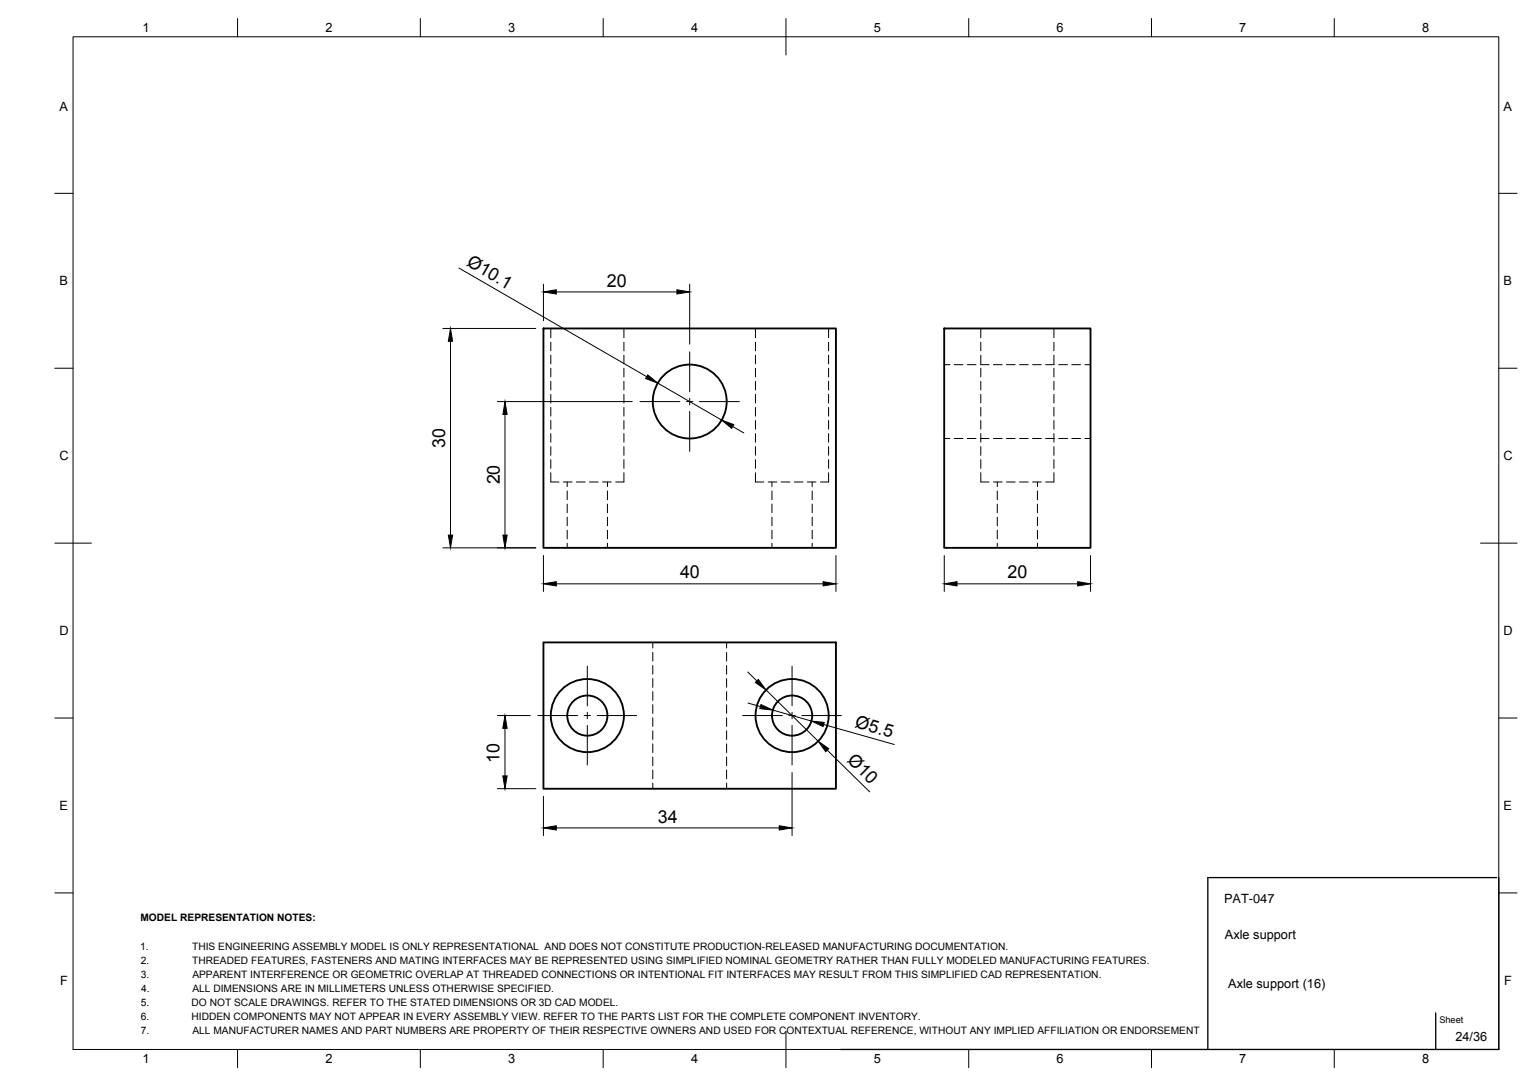
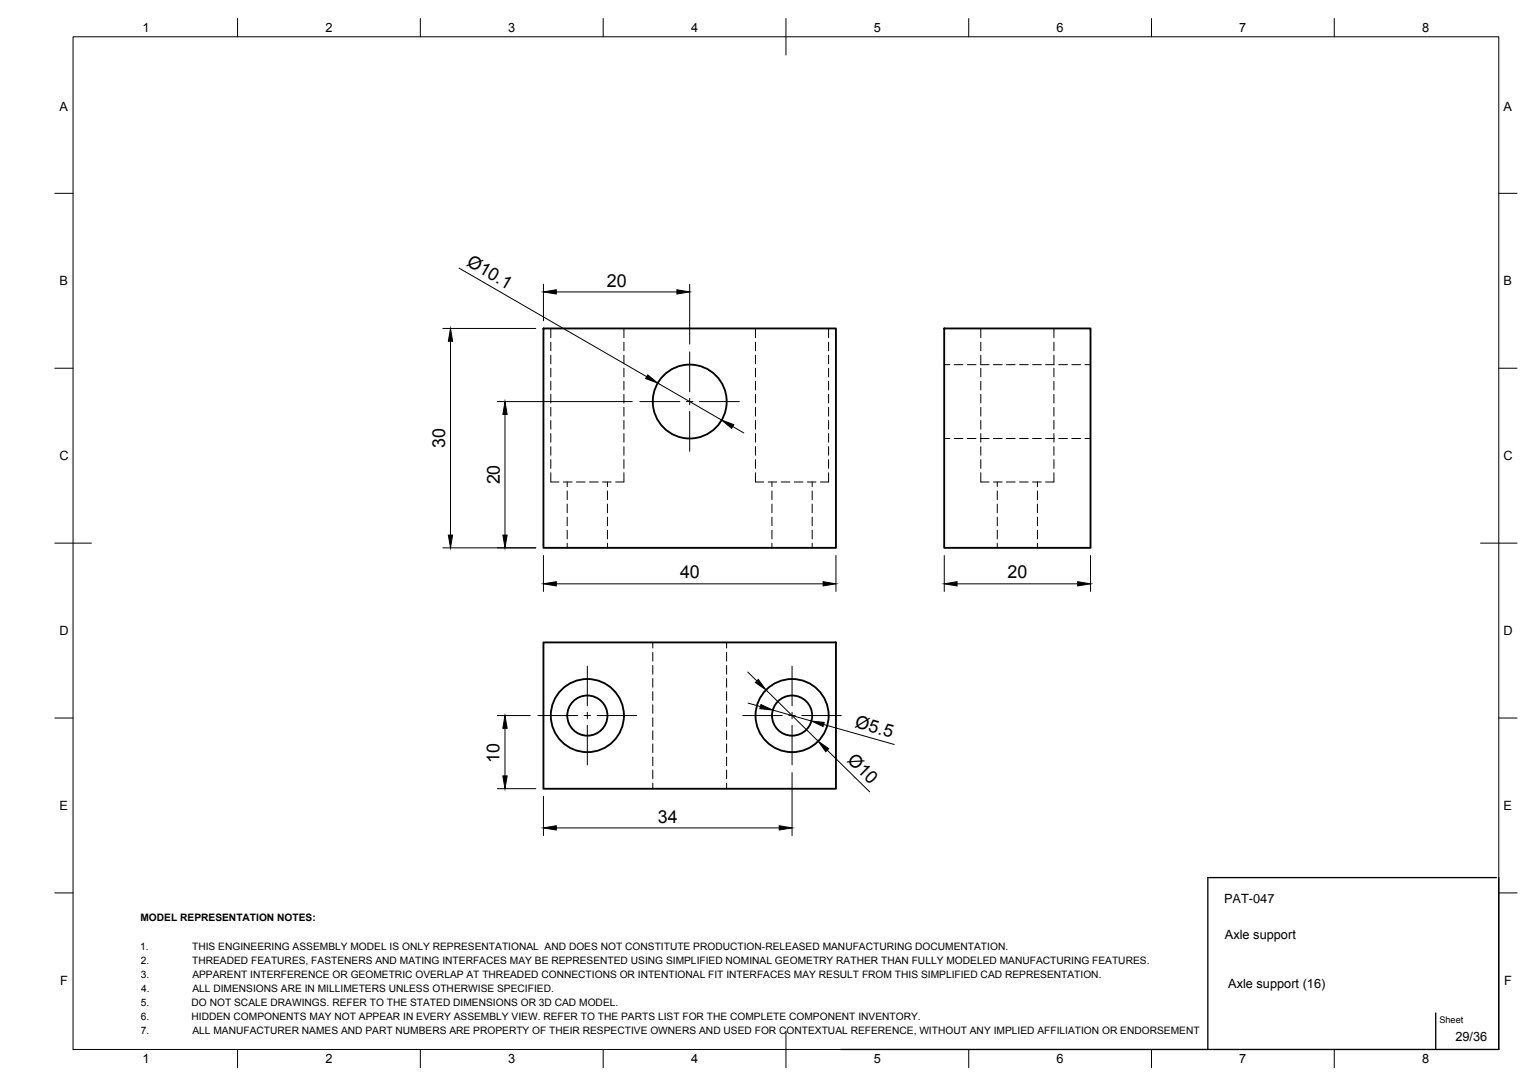
ISO-10303-21;
HEADER;
/* Generated by software containing ST-Developer
 * from STEP Tools, Inc. (www.steptools.com) 
 */

FILE_DESCRIPTION(
/* description */ ('Gravity roller conveyor section'),
/* implementation_level */ '2;1');

FILE_NAME(
/* name */ 'Axle support.step',
/* time_stamp */ '2026-11-02T07:43:02-08:00',
/* author */ (''),
/* organization */ (''),
/* preprocessor_version */ 'ST-DEVELOPER v20.2',
/* originating_system */ 'Autodesk Translation Framework v15.17.0.0',
/* authorisation */ '');

FILE_SCHEMA (('AUTOMOTIVE_DESIGN { 1 0 10303 214 3 1 1 }'));
ENDSEC;

DATA;
#10=MECHANICAL_DESIGN_GEOMETRIC_PRESENTATION_REPRESENTATION('',(#549),#13821);
#481=SHAPE_REPRESENTATION_RELATIONSHIP('SRR','None',#14019,#515);
#515=ADVANCED_BREP_SHAPE_REPRESENTATION('',(#589),#13806);
#549=STYLED_ITEM('',(#14192),#589);
#589=MANIFOLD_SOLID_BREP('Body1',#7649);
#666=FACE_BOUND('',#1765,.T.);
#667=FACE_BOUND('',#1768,.T.);
#668=FACE_BOUND('',#1773,.T.);
#669=FACE_BOUND('',#1776,.T.);
#670=FACE_BOUND('',#1779,.T.);
#671=FACE_BOUND('',#1780,.T.);
#672=FACE_BOUND('',#1782,.T.);
#673=FACE_BOUND('',#1783,.T.);
#931=PLANE('',#8445);
#932=PLANE('',#8450);
#933=PLANE('',#8459);
#934=PLANE('',#8460);
#935=PLANE('',#8461);
#936=PLANE('',#8462);
#937=PLANE('',#8463);
#938=PLANE('',#8464);
#1287=FACE_OUTER_BOUND('',#1763,.T.);
#1288=FACE_OUTER_BOUND('',#1764,.T.);
#1289=FACE_OUTER_BOUND('',#1766,.T.);
#1290=FACE_OUTER_BOUND('',#1767,.T.);
#1291=FACE_OUTER_BOUND('',#1769,.T.);
#1292=FACE_OUTER_BOUND('',#1770,.T.);
#1293=FACE_OUTER_BOUND('',#1771,.T.);
#1294=FACE_OUTER_BOUND('',#1772,.T.);
#1295=FACE_OUTER_BOUND('',#1774,.T.);
#1296=FACE_OUTER_BOUND('',#1775,.T.);
#1297=FACE_OUTER_BOUND('',#1777,.T.);
#1298=FACE_OUTER_BOUND('',#1778,.T.);
#1299=FACE_OUTER_BOUND('',#1781,.T.);
#1763=EDGE_LOOP('',(#6564,#6565,#6566,#6567));
#1764=EDGE_LOOP('',(#6568));
#1765=EDGE_LOOP('',(#6569));
#1766=EDGE_LOOP('',(#6570,#6571,#6572,#6573));
#1767=EDGE_LOOP('',(#6574));
#1768=EDGE_LOOP('',(#6575));
#1769=EDGE_LOOP('',(#6576,#6577,#6578,#6579));
#1770=EDGE_LOOP('',(#6580,#6581,#6582,#6583));
#1771=EDGE_LOOP('',(#6584,#6585,#6586,#6587));
#1772=EDGE_LOOP('',(#6588,#6589,#6590,#6591));
#1773=EDGE_LOOP('',(#6592));
#1774=EDGE_LOOP('',(#6593,#6594,#6595,#6596));
#1775=EDGE_LOOP('',(#6597,#6598,#6599,#6600));
#1776=EDGE_LOOP('',(#6601));
#1777=EDGE_LOOP('',(#6602,#6603,#6604,#6605));
#1778=EDGE_LOOP('',(#6606,#6607,#6608,#6609));
#1779=EDGE_LOOP('',(#6610));
#1780=EDGE_LOOP('',(#6611));
#1781=EDGE_LOOP('',(#6612,#6613,#6614,#6615));
#1782=EDGE_LOOP('',(#6616));
#1783=EDGE_LOOP('',(#6617));
#2519=LINE('',#12684,#3237);
#2520=LINE('',#12693,#3238);
#2521=LINE('',#12701,#3239);
#2522=LINE('',#12705,#3240);
#2523=LINE('',#12710,#3241);
#2524=LINE('',#12715,#3242);
#2525=LINE('',#12717,#3243);
#2526=LINE('',#12719,#3244);
#2527=LINE('',#12720,#3245);
#2528=LINE('',#12723,#3246);
#2529=LINE('',#12725,#3247);
#2530=LINE('',#12726,#3248);
#2531=LINE('',#12729,#3249);
#2532=LINE('',#12731,#3250);
#2533=LINE('',#12732,#3251);
#2534=LINE('',#12734,#3252);
#2535=LINE('',#12735,#3253);
#3237=VECTOR('',#10190,0.5);
#3238=VECTOR('',#10201,0.5);
#3239=VECTOR('',#10212,0.275);
#3240=VECTOR('',#10217,0.275);
#3241=VECTOR('',#10222,0.505);
#3242=VECTOR('',#10227,1.);
#3243=VECTOR('',#10228,1.);
#3244=VECTOR('',#10229,1.);
#3245=VECTOR('',#10230,1.);
#3246=VECTOR('',#10233,1.);
#3247=VECTOR('',#10234,1.);
#3248=VECTOR('',#10235,1.);
#3249=VECTOR('',#10238,1.);
#3250=VECTOR('',#10239,1.);
#3251=VECTOR('',#10240,1.);
#3252=VECTOR('',#10243,1.);
#3253=VECTOR('',#10244,1.);
#3464=CIRCLE('',#8443,0.5);
#3465=CIRCLE('',#8444,0.5);
#3466=CIRCLE('',#8446,0.275);
#3467=CIRCLE('',#8448,0.5);
#3468=CIRCLE('',#8449,0.5);
#3469=CIRCLE('',#8451,0.275);
#3470=CIRCLE('',#8453,0.275);
#3471=CIRCLE('',#8455,0.275);
#3472=CIRCLE('',#8457,0.505);
#3473=CIRCLE('',#8458,0.505);
#4042=VERTEX_POINT('',#12681);
#4043=VERTEX_POINT('',#12683);
#4044=VERTEX_POINT('',#12687);
#4045=VERTEX_POINT('',#12690);
#4046=VERTEX_POINT('',#12692);
#4047=VERTEX_POINT('',#12696);
#4048=VERTEX_POINT('',#12699);
#4049=VERTEX_POINT('',#12703);
#4050=VERTEX_POINT('',#12707);
#4051=VERTEX_POINT('',#12709);
#4052=VERTEX_POINT('',#12713);
#4053=VERTEX_POINT('',#12714);
#4054=VERTEX_POINT('',#12716);
#4055=VERTEX_POINT('',#12718);
#4056=VERTEX_POINT('',#12722);
#4057=VERTEX_POINT('',#12724);
#4058=VERTEX_POINT('',#12728);
#4059=VERTEX_POINT('',#12730);
#4919=EDGE_CURVE('',#4042,#4042,#3464,.T.);
#4920=EDGE_CURVE('',#4042,#4043,#2519,.T.);
#4921=EDGE_CURVE('',#4043,#4043,#3465,.T.);
#4922=EDGE_CURVE('',#4044,#4044,#3466,.T.);
#4923=EDGE_CURVE('',#4045,#4045,#3467,.T.);
#4924=EDGE_CURVE('',#4045,#4046,#2520,.T.);
#4925=EDGE_CURVE('',#4046,#4046,#3468,.T.);
#4926=EDGE_CURVE('',#4047,#4047,#3469,.T.);
#4927=EDGE_CURVE('',#4048,#4048,#3470,.T.);
#4928=EDGE_CURVE('',#4048,#4044,#2521,.T.);
#4929=EDGE_CURVE('',#4049,#4049,#3471,.T.);
#4930=EDGE_CURVE('',#4049,#4047,#2522,.T.);
#4931=EDGE_CURVE('',#4050,#4050,#3472,.T.);
#4932=EDGE_CURVE('',#4050,#4051,#2523,.T.);
#4933=EDGE_CURVE('',#4051,#4051,#3473,.T.);
#4934=EDGE_CURVE('',#4052,#4053,#2524,.T.);
#4935=EDGE_CURVE('',#4053,#4054,#2525,.T.);
#4936=EDGE_CURVE('',#4055,#4054,#2526,.T.);
#4937=EDGE_CURVE('',#4052,#4055,#2527,.T.);
#4938=EDGE_CURVE('',#4056,#4052,#2528,.T.);
#4939=EDGE_CURVE('',#4057,#4055,#2529,.T.);
#4940=EDGE_CURVE('',#4056,#4057,#2530,.T.);
#4941=EDGE_CURVE('',#4058,#4056,#2531,.T.);
#4942=EDGE_CURVE('',#4059,#4057,#2532,.T.);
#4943=EDGE_CURVE('',#4058,#4059,#2533,.T.);
#4944=EDGE_CURVE('',#4053,#4058,#2534,.T.);
#4945=EDGE_CURVE('',#4054,#4059,#2535,.T.);
#6564=ORIENTED_EDGE('',*,*,#4919,.F.);
#6565=ORIENTED_EDGE('',*,*,#4920,.T.);
#6566=ORIENTED_EDGE('',*,*,#4921,.F.);
#6567=ORIENTED_EDGE('',*,*,#4920,.F.);
#6568=ORIENTED_EDGE('',*,*,#4919,.T.);
#6569=ORIENTED_EDGE('',*,*,#4922,.F.);
#6570=ORIENTED_EDGE('',*,*,#4923,.F.);
#6571=ORIENTED_EDGE('',*,*,#4924,.T.);
#6572=ORIENTED_EDGE('',*,*,#4925,.F.);
#6573=ORIENTED_EDGE('',*,*,#4924,.F.);
#6574=ORIENTED_EDGE('',*,*,#4923,.T.);
#6575=ORIENTED_EDGE('',*,*,#4926,.F.);
#6576=ORIENTED_EDGE('',*,*,#4927,.F.);
#6577=ORIENTED_EDGE('',*,*,#4928,.T.);
#6578=ORIENTED_EDGE('',*,*,#4922,.T.);
#6579=ORIENTED_EDGE('',*,*,#4928,.F.);
#6580=ORIENTED_EDGE('',*,*,#4929,.F.);
#6581=ORIENTED_EDGE('',*,*,#4930,.T.);
#6582=ORIENTED_EDGE('',*,*,#4926,.T.);
#6583=ORIENTED_EDGE('',*,*,#4930,.F.);
#6584=ORIENTED_EDGE('',*,*,#4931,.F.);
#6585=ORIENTED_EDGE('',*,*,#4932,.T.);
#6586=ORIENTED_EDGE('',*,*,#4933,.F.);
#6587=ORIENTED_EDGE('',*,*,#4932,.F.);
#6588=ORIENTED_EDGE('',*,*,#4934,.T.);
#6589=ORIENTED_EDGE('',*,*,#4935,.T.);
#6590=ORIENTED_EDGE('',*,*,#4936,.F.);
#6591=ORIENTED_EDGE('',*,*,#4937,.F.);
#6592=ORIENTED_EDGE('',*,*,#4933,.T.);
#6593=ORIENTED_EDGE('',*,*,#4938,.T.);
#6594=ORIENTED_EDGE('',*,*,#4937,.T.);
#6595=ORIENTED_EDGE('',*,*,#4939,.F.);
#6596=ORIENTED_EDGE('',*,*,#4940,.F.);
#6597=ORIENTED_EDGE('',*,*,#4941,.T.);
#6598=ORIENTED_EDGE('',*,*,#4940,.T.);
#6599=ORIENTED_EDGE('',*,*,#4942,.F.);
#6600=ORIENTED_EDGE('',*,*,#4943,.F.);
#6601=ORIENTED_EDGE('',*,*,#4931,.T.);
#6602=ORIENTED_EDGE('',*,*,#4944,.T.);
#6603=ORIENTED_EDGE('',*,*,#4943,.T.);
#6604=ORIENTED_EDGE('',*,*,#4945,.F.);
#6605=ORIENTED_EDGE('',*,*,#4935,.F.);
#6606=ORIENTED_EDGE('',*,*,#4945,.T.);
#6607=ORIENTED_EDGE('',*,*,#4942,.T.);
#6608=ORIENTED_EDGE('',*,*,#4939,.T.);
#6609=ORIENTED_EDGE('',*,*,#4936,.T.);
#6610=ORIENTED_EDGE('',*,*,#4921,.T.);
#6611=ORIENTED_EDGE('',*,*,#4925,.T.);
#6612=ORIENTED_EDGE('',*,*,#4944,.F.);
#6613=ORIENTED_EDGE('',*,*,#4934,.F.);
#6614=ORIENTED_EDGE('',*,*,#4938,.F.);
#6615=ORIENTED_EDGE('',*,*,#4941,.F.);
#6616=ORIENTED_EDGE('',*,*,#4927,.T.);
#6617=ORIENTED_EDGE('',*,*,#4929,.T.);
#7173=CYLINDRICAL_SURFACE('',#8442,0.5);
#7174=CYLINDRICAL_SURFACE('',#8447,0.5);
#7175=CYLINDRICAL_SURFACE('',#8452,0.275);
#7176=CYLINDRICAL_SURFACE('',#8454,0.275);
#7177=CYLINDRICAL_SURFACE('',#8456,0.505);
#7488=ADVANCED_FACE('',(#1287),#7173,.F.);
#7489=ADVANCED_FACE('',(#1288,#666),#931,.T.);
#7490=ADVANCED_FACE('',(#1289),#7174,.F.);
#7491=ADVANCED_FACE('',(#1290,#667),#932,.T.);
#7492=ADVANCED_FACE('',(#1291),#7175,.F.);
#7493=ADVANCED_FACE('',(#1292),#7176,.F.);
#7494=ADVANCED_FACE('',(#1293),#7177,.F.);
#7495=ADVANCED_FACE('',(#1294,#668),#933,.T.);
#7496=ADVANCED_FACE('',(#1295),#934,.T.);
#7497=ADVANCED_FACE('',(#1296,#669),#935,.T.);
#7498=ADVANCED_FACE('',(#1297),#936,.T.);
#7499=ADVANCED_FACE('',(#1298,#670,#671),#937,.T.);
#7500=ADVANCED_FACE('',(#1299,#672,#673),#938,.F.);
#7649=CLOSED_SHELL('',(#7488,#7489,#7490,#7491,#7492,#7493,#7494,#7495,
#7496,#7497,#7498,#7499,#7500));
#8441=AXIS2_PLACEMENT_3D('',#12679,#10184,#10185);
#8442=AXIS2_PLACEMENT_3D('',#12680,#10186,#10187);
#8443=AXIS2_PLACEMENT_3D('',#12682,#10188,#10189);
#8444=AXIS2_PLACEMENT_3D('',#12685,#10191,#10192);
#8445=AXIS2_PLACEMENT_3D('',#12686,#10193,#10194);
#8446=AXIS2_PLACEMENT_3D('',#12688,#10195,#10196);
#8447=AXIS2_PLACEMENT_3D('',#12689,#10197,#10198);
#8448=AXIS2_PLACEMENT_3D('',#12691,#10199,#10200);
#8449=AXIS2_PLACEMENT_3D('',#12694,#10202,#10203);
#8450=AXIS2_PLACEMENT_3D('',#12695,#10204,#10205);
#8451=AXIS2_PLACEMENT_3D('',#12697,#10206,#10207);
#8452=AXIS2_PLACEMENT_3D('',#12698,#10208,#10209);
#8453=AXIS2_PLACEMENT_3D('',#12700,#10210,#10211);
#8454=AXIS2_PLACEMENT_3D('',#12702,#10213,#10214);
#8455=AXIS2_PLACEMENT_3D('',#12704,#10215,#10216);
#8456=AXIS2_PLACEMENT_3D('',#12706,#10218,#10219);
#8457=AXIS2_PLACEMENT_3D('',#12708,#10220,#10221);
#8458=AXIS2_PLACEMENT_3D('',#12711,#10223,#10224);
#8459=AXIS2_PLACEMENT_3D('',#12712,#10225,#10226);
#8460=AXIS2_PLACEMENT_3D('',#12721,#10231,#10232);
#8461=AXIS2_PLACEMENT_3D('',#12727,#10236,#10237);
#8462=AXIS2_PLACEMENT_3D('',#12733,#10241,#10242);
#8463=AXIS2_PLACEMENT_3D('',#12736,#10245,#10246);
#8464=AXIS2_PLACEMENT_3D('',#12737,#10247,#10248);
#10184=DIRECTION('axis',(0.,0.,1.));
#10185=DIRECTION('refdir',(1.,0.,0.));
#10186=DIRECTION('center_axis',(0.,0.,1.));
#10187=DIRECTION('ref_axis',(1.,0.,0.));
#10188=DIRECTION('center_axis',(0.,0.,1.));
#10189=DIRECTION('ref_axis',(1.,0.,0.));
#10190=DIRECTION('',(0.,0.,1.));
#10191=DIRECTION('center_axis',(0.,0.,-1.));
#10192=DIRECTION('ref_axis',(1.,0.,0.));
#10193=DIRECTION('center_axis',(0.,0.,1.));
#10194=DIRECTION('ref_axis',(1.,0.,0.));
#10195=DIRECTION('center_axis',(0.,0.,1.));
#10196=DIRECTION('ref_axis',(1.,0.,0.));
#10197=DIRECTION('center_axis',(0.,0.,1.));
#10198=DIRECTION('ref_axis',(1.,0.,0.));
#10199=DIRECTION('center_axis',(0.,0.,1.));
#10200=DIRECTION('ref_axis',(1.,0.,0.));
#10201=DIRECTION('',(0.,0.,1.));
#10202=DIRECTION('center_axis',(0.,0.,-1.));
#10203=DIRECTION('ref_axis',(1.,0.,0.));
#10204=DIRECTION('center_axis',(0.,0.,1.));
#10205=DIRECTION('ref_axis',(1.,0.,0.));
#10206=DIRECTION('center_axis',(0.,0.,1.));
#10207=DIRECTION('ref_axis',(1.,0.,0.));
#10208=DIRECTION('center_axis',(0.,0.,1.));
#10209=DIRECTION('ref_axis',(1.,0.,0.));
#10210=DIRECTION('center_axis',(0.,0.,1.));
#10211=DIRECTION('ref_axis',(1.,0.,0.));
#10212=DIRECTION('',(0.,0.,1.));
#10213=DIRECTION('center_axis',(0.,0.,1.));
#10214=DIRECTION('ref_axis',(1.,0.,0.));
#10215=DIRECTION('center_axis',(0.,0.,1.));
#10216=DIRECTION('ref_axis',(1.,0.,0.));
#10217=DIRECTION('',(0.,0.,1.));
#10218=DIRECTION('center_axis',(0.,1.,0.));
#10219=DIRECTION('ref_axis',(1.,0.,0.));
#10220=DIRECTION('center_axis',(0.,1.,0.));
#10221=DIRECTION('ref_axis',(1.,0.,0.));
#10222=DIRECTION('',(0.,1.,0.));
#10223=DIRECTION('center_axis',(0.,-1.,0.));
#10224=DIRECTION('ref_axis',(1.,0.,0.));
#10225=DIRECTION('center_axis',(0.,1.,0.));
#10226=DIRECTION('ref_axis',(-1.,0.,0.));
#10227=DIRECTION('',(-1.,0.,0.));
#10228=DIRECTION('',(0.,0.,1.));
#10229=DIRECTION('',(-1.,0.,0.));
#10230=DIRECTION('',(0.,0.,1.));
#10231=DIRECTION('center_axis',(1.,0.,0.));
#10232=DIRECTION('ref_axis',(0.,1.,0.));
#10233=DIRECTION('',(0.,1.,0.));
#10234=DIRECTION('',(0.,1.,0.));
#10235=DIRECTION('',(0.,0.,1.));
#10236=DIRECTION('center_axis',(0.,-1.,0.));
#10237=DIRECTION('ref_axis',(1.,0.,0.));
#10238=DIRECTION('',(1.,0.,0.));
#10239=DIRECTION('',(1.,0.,0.));
#10240=DIRECTION('',(0.,0.,1.));
#10241=DIRECTION('center_axis',(-1.,0.,0.));
#10242=DIRECTION('ref_axis',(0.,-1.,0.));
#10243=DIRECTION('',(0.,-1.,0.));
#10244=DIRECTION('',(0.,-1.,0.));
#10245=DIRECTION('center_axis',(0.,0.,1.));
#10246=DIRECTION('ref_axis',(1.,0.,0.));
#10247=DIRECTION('center_axis',(0.,0.,1.));
#10248=DIRECTION('ref_axis',(1.,0.,0.));
#12679=CARTESIAN_POINT('',(0.,0.,0.));
#12680=CARTESIAN_POINT('Origin',(1.6,-2.,6.9));
#12681=CARTESIAN_POINT('',(1.1,-2.,6.9));
#12682=CARTESIAN_POINT('Origin',(1.6,-2.,6.9));
#12683=CARTESIAN_POINT('',(1.1,-2.,9.));
#12684=CARTESIAN_POINT('',(1.1,-2.,6.9));
#12685=CARTESIAN_POINT('Origin',(1.6,-2.,9.));
#12686=CARTESIAN_POINT('Origin',(1.6,-2.,6.9));
#12687=CARTESIAN_POINT('',(1.325,-2.,6.9));
#12688=CARTESIAN_POINT('Origin',(1.6,-2.,6.9));
#12689=CARTESIAN_POINT('Origin',(4.4,-2.,6.9));
#12690=CARTESIAN_POINT('',(3.9,-2.,6.9));
#12691=CARTESIAN_POINT('Origin',(4.4,-2.,6.9));
#12692=CARTESIAN_POINT('',(3.9,-2.,9.));
#12693=CARTESIAN_POINT('',(3.9,-2.,6.9));
#12694=CARTESIAN_POINT('Origin',(4.4,-2.,9.));
#12695=CARTESIAN_POINT('Origin',(4.4,-2.,6.9));
#12696=CARTESIAN_POINT('',(4.125,-2.,6.9));
#12697=CARTESIAN_POINT('Origin',(4.4,-2.,6.9));
#12698=CARTESIAN_POINT('Origin',(1.6,-2.,5.9));
#12699=CARTESIAN_POINT('',(1.325,-2.,6.));
#12700=CARTESIAN_POINT('Origin',(1.6,-2.,6.));
#12701=CARTESIAN_POINT('',(1.325,-2.,5.9));
#12702=CARTESIAN_POINT('Origin',(4.4,-2.,5.9));
#12703=CARTESIAN_POINT('',(4.125,-2.,6.));
#12704=CARTESIAN_POINT('Origin',(4.4,-2.,6.));
#12705=CARTESIAN_POINT('',(4.125,-2.,5.9));
#12706=CARTESIAN_POINT('Origin',(3.,-3.1,8.));
#12707=CARTESIAN_POINT('',(2.495,-3.,8.));
#12708=CARTESIAN_POINT('Origin',(3.,-3.,8.));
#12709=CARTESIAN_POINT('',(2.495,-1.,8.));
#12710=CARTESIAN_POINT('',(2.495,-3.1,8.));
#12711=CARTESIAN_POINT('Origin',(3.,-1.,8.));
#12712=CARTESIAN_POINT('Origin',(5.,-1.,6.));
#12713=CARTESIAN_POINT('',(5.,-1.,6.));
#12714=CARTESIAN_POINT('',(1.,-1.,6.));
#12715=CARTESIAN_POINT('',(5.,-1.,6.));
#12716=CARTESIAN_POINT('',(1.,-1.,9.));
#12717=CARTESIAN_POINT('',(1.,-1.,6.));
#12718=CARTESIAN_POINT('',(5.,-1.,9.));
#12719=CARTESIAN_POINT('',(5.,-1.,9.));
#12720=CARTESIAN_POINT('',(5.,-1.,6.));
#12721=CARTESIAN_POINT('Origin',(5.,-3.,6.));
#12722=CARTESIAN_POINT('',(5.,-3.,6.));
#12723=CARTESIAN_POINT('',(5.,-3.,6.));
#12724=CARTESIAN_POINT('',(5.,-3.,9.));
#12725=CARTESIAN_POINT('',(5.,-3.,9.));
#12726=CARTESIAN_POINT('',(5.,-3.,6.));
#12727=CARTESIAN_POINT('Origin',(1.,-3.,6.));
#12728=CARTESIAN_POINT('',(1.,-3.,6.));
#12729=CARTESIAN_POINT('',(1.,-3.,6.));
#12730=CARTESIAN_POINT('',(1.,-3.,9.));
#12731=CARTESIAN_POINT('',(1.,-3.,9.));
#12732=CARTESIAN_POINT('',(1.,-3.,6.));
#12733=CARTESIAN_POINT('Origin',(1.,-1.,6.));
#12734=CARTESIAN_POINT('',(1.,-1.,6.));
#12735=CARTESIAN_POINT('',(1.,-1.,9.));
#12736=CARTESIAN_POINT('Origin',(3.,-2.,9.));
#12737=CARTESIAN_POINT('Origin',(3.,-2.,6.));
#13767=UNCERTAINTY_MEASURE_WITH_UNIT(LENGTH_MEASURE(0.001),#13822,
'DISTANCE_ACCURACY_VALUE',
'Maximum model space distance between geometric entities at asserted c
onnectivities');
#13782=UNCERTAINTY_MEASURE_WITH_UNIT(LENGTH_MEASURE(0.001),#13822,
'DISTANCE_ACCURACY_VALUE',
'Maximum model space distance between geometric entities at asserted c
onnectivities');
#13806=(
GEOMETRIC_REPRESENTATION_CONTEXT(3)
GLOBAL_UNCERTAINTY_ASSIGNED_CONTEXT((#13767))
GLOBAL_UNIT_ASSIGNED_CONTEXT((#13822,#13824,#13825))
REPRESENTATION_CONTEXT('','3D')
);
#13821=(
GEOMETRIC_REPRESENTATION_CONTEXT(3)
GLOBAL_UNCERTAINTY_ASSIGNED_CONTEXT((#13782))
GLOBAL_UNIT_ASSIGNED_CONTEXT((#13822,#13824,#13825))
REPRESENTATION_CONTEXT('','3D')
);
#13822=(
LENGTH_UNIT()
NAMED_UNIT(*)
SI_UNIT(.CENTI.,.METRE.)
);
#13824=(
NAMED_UNIT(*)
PLANE_ANGLE_UNIT()
SI_UNIT($,.RADIAN.)
);
#13825=(
NAMED_UNIT(*)
SI_UNIT($,.STERADIAN.)
SOLID_ANGLE_UNIT()
);
#13849=SHAPE_DEFINITION_REPRESENTATION(#13887,#14019);
#13887=PRODUCT_DEFINITION_SHAPE('',$,#14058);
#14019=SHAPE_REPRESENTATION('',(#8441),#13806);
#14034=PRODUCT_DEFINITION_CONTEXT('part definition',#14150,'design');
#14058=PRODUCT_DEFINITION('Axle support','Axle support',#14096,#14034);
#14096=PRODUCT_DEFINITION_FORMATION('',$,#14175);
#14150=APPLICATION_CONTEXT(
'Core Data for Automotive Mechanical Design Process');
#14151=PRODUCT_CONTEXT('part definition',#14150,'mechanical');
#14175=PRODUCT('Axle support','Axle support','Axle support',(#14151));
#14192=PRESENTATION_STYLE_ASSIGNMENT((#14197));
#14197=SURFACE_STYLE_USAGE(.BOTH.,#14202);
#14202=SURFACE_SIDE_STYLE('',(#14207));
#14207=SURFACE_STYLE_FILL_AREA(#14212);
#14212=FILL_AREA_STYLE('CAD Library Painted - Engineering blue',(#14217));
#14217=FILL_AREA_STYLE_COLOUR('CAD Library Painted - Engineering blue',
#14222);
#14222=COLOUR_RGB('CAD Library Painted - Engineering blue',0.12156862745098,
0.356862745098039,0.6);
ENDSEC;
END-ISO-10303-21;
